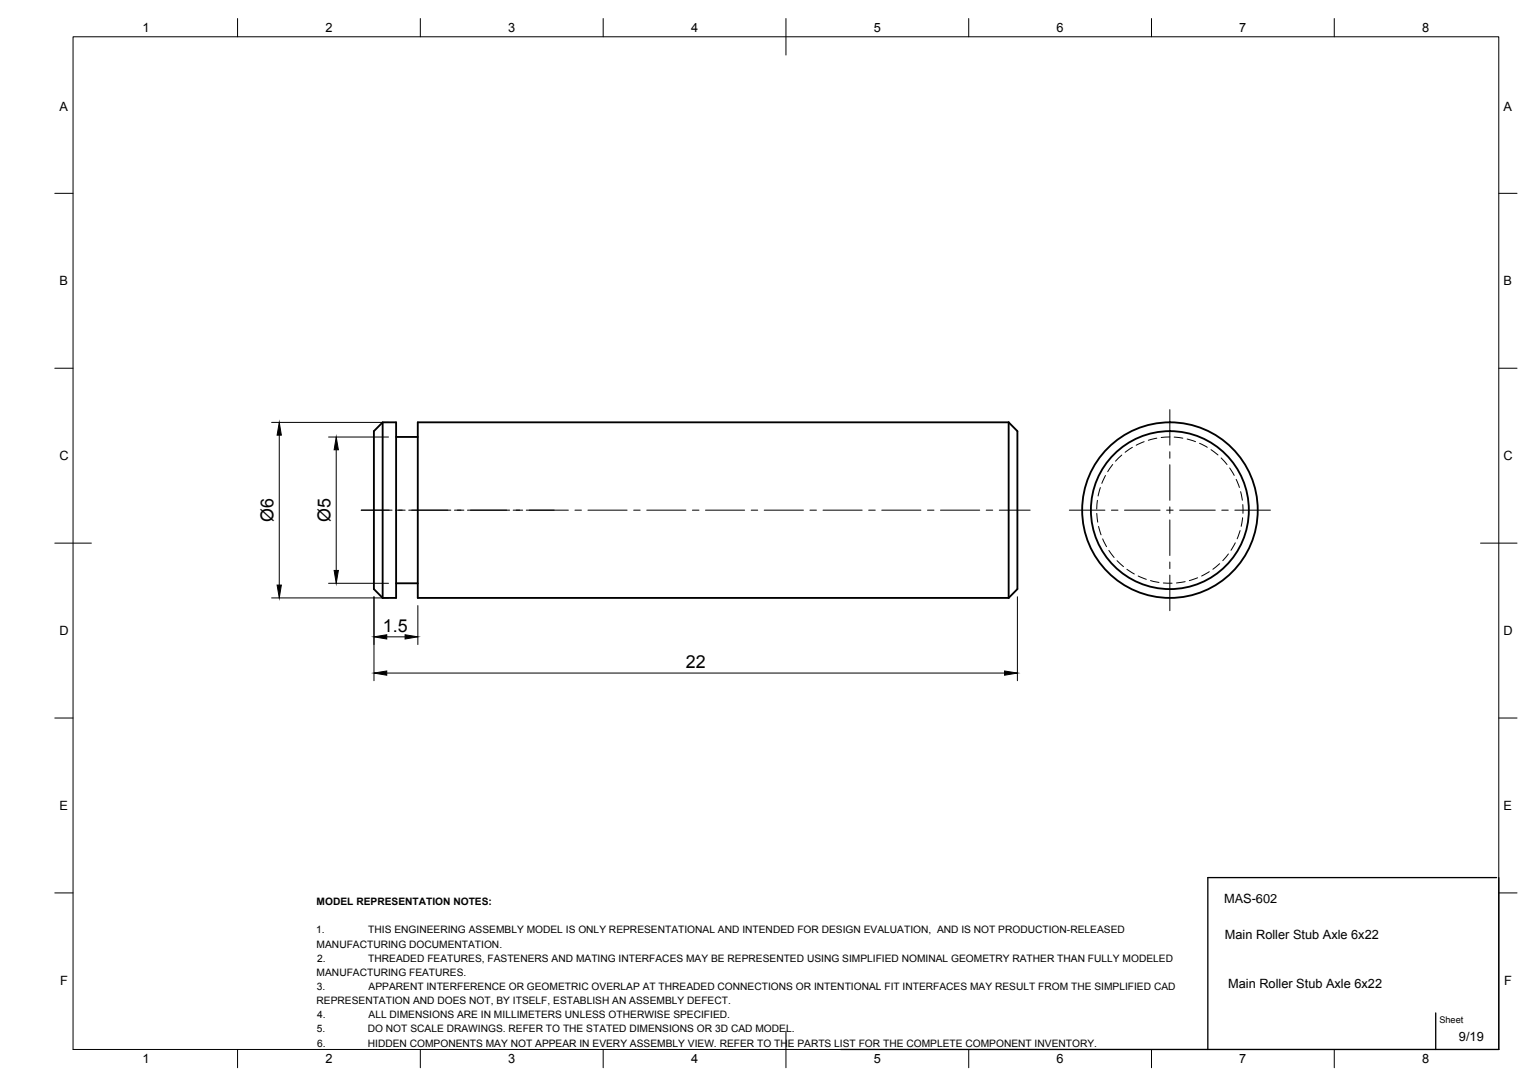
ISO-10303-21;
HEADER;
/* Generated by software containing ST-Developer
 * from STEP Tools, Inc. (www.steptools.com) 
 */

FILE_DESCRIPTION(
/* description */ (''),
/* implementation_level */ '2;1');

FILE_NAME(
/* name */ 'Main Roller Stub Axle 6x22.step',
/* time_stamp */ '2026-10-15T14:42:47-07:00',
/* author */ (''),
/* organization */ (''),
/* preprocessor_version */ 'ST-DEVELOPER v20.2',
/* originating_system */ 'Autodesk Translation Framework v15.15.0.0',
/* authorisation */ '');

FILE_SCHEMA (('AUTOMOTIVE_DESIGN { 1 0 10303 214 3 1 1 }'));
ENDSEC;

DATA;
#10=MECHANICAL_DESIGN_GEOMETRIC_PRESENTATION_REPRESENTATION('',(#246),#85789);
#185=CONICAL_SURFACE('',#10744,0.285,0.785398163397449);
#186=CONICAL_SURFACE('',#10756,0.285,0.785398163397444);
#210=SHAPE_REPRESENTATION_RELATIONSHIP('SRR','None',#85875,#228);
#228=ADVANCED_BREP_SHAPE_REPRESENTATION('',(#264),#85783);
#246=STYLED_ITEM('',(#85974),#264);
#264=MANIFOLD_SOLID_BREP('Body1',#9893);
#469=FACE_BOUND('',#3398,.T.);
#470=FACE_BOUND('',#3401,.T.);
#1167=PLANE('',#10742);
#1168=PLANE('',#10748);
#1169=PLANE('',#10752);
#1170=PLANE('',#10758);
#1650=LINE('',#77818,#2186);
#1651=LINE('',#77822,#2187);
#1652=LINE('',#77829,#2188);
#1653=LINE('',#77836,#2189);
#1654=LINE('',#77839,#2190);
#2186=VECTOR('',#12706,0.285);
#2187=VECTOR('',#12711,0.3);
#2188=VECTOR('',#12720,0.25);
#2189=VECTOR('',#12729,0.3);
#2190=VECTOR('',#12732,0.285);
#2358=CYLINDRICAL_SURFACE('',#10746,0.3);
#2359=CYLINDRICAL_SURFACE('',#10750,0.25);
#2360=CYLINDRICAL_SURFACE('',#10754,0.3);
#2810=FACE_OUTER_BOUND('',#3394,.T.);
#2811=FACE_OUTER_BOUND('',#3395,.T.);
#2812=FACE_OUTER_BOUND('',#3396,.T.);
#2813=FACE_OUTER_BOUND('',#3397,.T.);
#2814=FACE_OUTER_BOUND('',#3399,.T.);
#2815=FACE_OUTER_BOUND('',#3400,.T.);
#2816=FACE_OUTER_BOUND('',#3402,.T.);
#2817=FACE_OUTER_BOUND('',#3403,.T.);
#2818=FACE_OUTER_BOUND('',#3404,.T.);
#3394=EDGE_LOOP('',(#8837));
#3395=EDGE_LOOP('',(#8838,#8839,#8840,#8841));
#3396=EDGE_LOOP('',(#8842,#8843,#8844,#8845));
#3397=EDGE_LOOP('',(#8846));
#3398=EDGE_LOOP('',(#8847));
#3399=EDGE_LOOP('',(#8848,#8849,#8850,#8851));
#3400=EDGE_LOOP('',(#8852));
#3401=EDGE_LOOP('',(#8853));
#3402=EDGE_LOOP('',(#8854,#8855,#8856,#8857));
#3403=EDGE_LOOP('',(#8858,#8859,#8860,#8861));
#3404=EDGE_LOOP('',(#8862));
#3804=CIRCLE('',#10743,0.27);
#3805=CIRCLE('',#10745,0.3);
#3806=CIRCLE('',#10747,0.3);
#3807=CIRCLE('',#10749,0.25);
#3808=CIRCLE('',#10751,0.25);
#3809=CIRCLE('',#10753,0.3);
#3810=CIRCLE('',#10755,0.3);
#3811=CIRCLE('',#10757,0.27);
#4741=VERTEX_POINT('',#77813);
#4742=VERTEX_POINT('',#77816);
#4743=VERTEX_POINT('',#77820);
#4744=VERTEX_POINT('',#77824);
#4745=VERTEX_POINT('',#77827);
#4746=VERTEX_POINT('',#77831);
#4747=VERTEX_POINT('',#77834);
#4748=VERTEX_POINT('',#77838);
#6146=EDGE_CURVE('',#4741,#4741,#3804,.T.);
#6147=EDGE_CURVE('',#4742,#4742,#3805,.T.);
#6148=EDGE_CURVE('',#4742,#4741,#1650,.T.);
#6149=EDGE_CURVE('',#4743,#4743,#3806,.T.);
#6150=EDGE_CURVE('',#4743,#4742,#1651,.T.);
#6151=EDGE_CURVE('',#4744,#4744,#3807,.T.);
#6152=EDGE_CURVE('',#4745,#4745,#3808,.T.);
#6153=EDGE_CURVE('',#4745,#4744,#1652,.T.);
#6154=EDGE_CURVE('',#4746,#4746,#3809,.T.);
#6155=EDGE_CURVE('',#4747,#4747,#3810,.T.);
#6156=EDGE_CURVE('',#4747,#4746,#1653,.T.);
#6157=EDGE_CURVE('',#4747,#4748,#1654,.T.);
#6158=EDGE_CURVE('',#4748,#4748,#3811,.T.);
#8837=ORIENTED_EDGE('',*,*,#6146,.F.);
#8838=ORIENTED_EDGE('',*,*,#6147,.F.);
#8839=ORIENTED_EDGE('',*,*,#6148,.T.);
#8840=ORIENTED_EDGE('',*,*,#6146,.T.);
#8841=ORIENTED_EDGE('',*,*,#6148,.F.);
#8842=ORIENTED_EDGE('',*,*,#6149,.F.);
#8843=ORIENTED_EDGE('',*,*,#6150,.T.);
#8844=ORIENTED_EDGE('',*,*,#6147,.T.);
#8845=ORIENTED_EDGE('',*,*,#6150,.F.);
#8846=ORIENTED_EDGE('',*,*,#6149,.T.);
#8847=ORIENTED_EDGE('',*,*,#6151,.F.);
#8848=ORIENTED_EDGE('',*,*,#6152,.F.);
#8849=ORIENTED_EDGE('',*,*,#6153,.T.);
#8850=ORIENTED_EDGE('',*,*,#6151,.T.);
#8851=ORIENTED_EDGE('',*,*,#6153,.F.);
#8852=ORIENTED_EDGE('',*,*,#6154,.F.);
#8853=ORIENTED_EDGE('',*,*,#6152,.T.);
#8854=ORIENTED_EDGE('',*,*,#6155,.F.);
#8855=ORIENTED_EDGE('',*,*,#6156,.T.);
#8856=ORIENTED_EDGE('',*,*,#6154,.T.);
#8857=ORIENTED_EDGE('',*,*,#6156,.F.);
#8858=ORIENTED_EDGE('',*,*,#6155,.T.);
#8859=ORIENTED_EDGE('',*,*,#6157,.T.);
#8860=ORIENTED_EDGE('',*,*,#6158,.F.);
#8861=ORIENTED_EDGE('',*,*,#6157,.F.);
#8862=ORIENTED_EDGE('',*,*,#6158,.T.);
#9788=ADVANCED_FACE('',(#2810),#1167,.T.);
#9789=ADVANCED_FACE('',(#2811),#185,.T.);
#9790=ADVANCED_FACE('',(#2812),#2358,.T.);
#9791=ADVANCED_FACE('',(#2813,#469),#1168,.T.);
#9792=ADVANCED_FACE('',(#2814),#2359,.T.);
#9793=ADVANCED_FACE('',(#2815,#470),#1169,.T.);
#9794=ADVANCED_FACE('',(#2816),#2360,.T.);
#9795=ADVANCED_FACE('',(#2817),#186,.T.);
#9796=ADVANCED_FACE('',(#2818),#1170,.T.);
#9893=CLOSED_SHELL('',(#9788,#9789,#9790,#9791,#9792,#9793,#9794,#9795,
#9796));
#10741=AXIS2_PLACEMENT_3D('',#77811,#12696,#12697);
#10742=AXIS2_PLACEMENT_3D('',#77812,#12698,#12699);
#10743=AXIS2_PLACEMENT_3D('',#77814,#12700,#12701);
#10744=AXIS2_PLACEMENT_3D('',#77815,#12702,#12703);
#10745=AXIS2_PLACEMENT_3D('',#77817,#12704,#12705);
#10746=AXIS2_PLACEMENT_3D('',#77819,#12707,#12708);
#10747=AXIS2_PLACEMENT_3D('',#77821,#12709,#12710);
#10748=AXIS2_PLACEMENT_3D('',#77823,#12712,#12713);
#10749=AXIS2_PLACEMENT_3D('',#77825,#12714,#12715);
#10750=AXIS2_PLACEMENT_3D('',#77826,#12716,#12717);
#10751=AXIS2_PLACEMENT_3D('',#77828,#12718,#12719);
#10752=AXIS2_PLACEMENT_3D('',#77830,#12721,#12722);
#10753=AXIS2_PLACEMENT_3D('',#77832,#12723,#12724);
#10754=AXIS2_PLACEMENT_3D('',#77833,#12725,#12726);
#10755=AXIS2_PLACEMENT_3D('',#77835,#12727,#12728);
#10756=AXIS2_PLACEMENT_3D('',#77837,#12730,#12731);
#10757=AXIS2_PLACEMENT_3D('',#77840,#12733,#12734);
#10758=AXIS2_PLACEMENT_3D('',#77841,#12735,#12736);
#12696=DIRECTION('axis',(0.,0.,1.));
#12697=DIRECTION('refdir',(1.,0.,0.));
#12698=DIRECTION('center_axis',(-1.,0.,0.));
#12699=DIRECTION('ref_axis',(0.,0.,1.));
#12700=DIRECTION('center_axis',(1.,0.,0.));
#12701=DIRECTION('ref_axis',(0.,0.,-1.));
#12702=DIRECTION('center_axis',(1.,0.,0.));
#12703=DIRECTION('ref_axis',(0.,1.,0.));
#12704=DIRECTION('center_axis',(1.,0.,0.));
#12705=DIRECTION('ref_axis',(0.,0.,-1.));
#12706=DIRECTION('',(-0.707106781186547,0.707106781186548,8.65956056235494E-17));
#12707=DIRECTION('center_axis',(1.,0.,0.));
#12708=DIRECTION('ref_axis',(0.,1.,0.));
#12709=DIRECTION('center_axis',(1.,0.,0.));
#12710=DIRECTION('ref_axis',(0.,0.,-1.));
#12711=DIRECTION('',(-1.,0.,0.));
#12712=DIRECTION('center_axis',(1.,0.,0.));
#12713=DIRECTION('ref_axis',(0.,0.,-1.));
#12714=DIRECTION('center_axis',(1.,0.,0.));
#12715=DIRECTION('ref_axis',(0.,0.,-1.));
#12716=DIRECTION('center_axis',(1.,0.,0.));
#12717=DIRECTION('ref_axis',(0.,1.,0.));
#12718=DIRECTION('center_axis',(1.,0.,0.));
#12719=DIRECTION('ref_axis',(0.,0.,-1.));
#12720=DIRECTION('',(-1.,0.,0.));
#12721=DIRECTION('center_axis',(-1.,0.,0.));
#12722=DIRECTION('ref_axis',(0.,0.,1.));
#12723=DIRECTION('center_axis',(1.,0.,0.));
#12724=DIRECTION('ref_axis',(0.,0.,-1.));
#12725=DIRECTION('center_axis',(1.,0.,0.));
#12726=DIRECTION('ref_axis',(0.,1.,0.));
#12727=DIRECTION('center_axis',(1.,0.,0.));
#12728=DIRECTION('ref_axis',(0.,0.,-1.));
#12729=DIRECTION('',(-1.,0.,0.));
#12730=DIRECTION('center_axis',(-1.,0.,0.));
#12731=DIRECTION('ref_axis',(0.,1.,0.));
#12732=DIRECTION('',(0.707106781186551,0.707106781186544,-8.6595605623549E-17));
#12733=DIRECTION('center_axis',(1.,0.,0.));
#12734=DIRECTION('ref_axis',(0.,0.,-1.));
#12735=DIRECTION('center_axis',(1.,0.,0.));
#12736=DIRECTION('ref_axis',(0.,0.,-1.));
#77811=CARTESIAN_POINT('',(0.,0.,0.));
#77812=CARTESIAN_POINT('Origin',(0.55,0.27,0.));
#77813=CARTESIAN_POINT('',(0.55,-0.27,-3.30654635769785E-17));
#77814=CARTESIAN_POINT('Origin',(0.55,0.,0.));
#77815=CARTESIAN_POINT('Origin',(0.565,0.,0.));
#77816=CARTESIAN_POINT('',(0.58,-0.3,-3.67394039744206E-17));
#77817=CARTESIAN_POINT('Origin',(0.58,0.,0.));
#77818=CARTESIAN_POINT('',(0.565,-0.285,-3.49024337756996E-17));
#77819=CARTESIAN_POINT('Origin',(1.59,0.,0.));
#77820=CARTESIAN_POINT('',(2.6,-0.3,-3.67394039744206E-17));
#77821=CARTESIAN_POINT('Origin',(2.6,0.,0.));
#77822=CARTESIAN_POINT('',(1.59,-0.3,-3.67394039744206E-17));
#77823=CARTESIAN_POINT('Origin',(2.6,0.25,0.));
#77824=CARTESIAN_POINT('',(2.6,-0.25,-3.06161699786838E-17));
#77825=CARTESIAN_POINT('Origin',(2.6,0.,0.));
#77826=CARTESIAN_POINT('Origin',(2.637,0.,0.));
#77827=CARTESIAN_POINT('',(2.674,-0.25,-3.06161699786838E-17));
#77828=CARTESIAN_POINT('Origin',(2.674,0.,0.));
#77829=CARTESIAN_POINT('',(2.637,-0.25,-3.06161699786838E-17));
#77830=CARTESIAN_POINT('Origin',(2.674,0.3,0.));
#77831=CARTESIAN_POINT('',(2.674,-0.3,-3.67394039744206E-17));
#77832=CARTESIAN_POINT('Origin',(2.674,0.,0.));
#77833=CARTESIAN_POINT('Origin',(2.697,0.,0.));
#77834=CARTESIAN_POINT('',(2.72,-0.3,-3.67394039744206E-17));
#77835=CARTESIAN_POINT('Origin',(2.72,0.,0.));
#77836=CARTESIAN_POINT('',(2.697,-0.3,-3.67394039744206E-17));
#77837=CARTESIAN_POINT('Origin',(2.735,0.,0.));
#77838=CARTESIAN_POINT('',(2.75,-0.27,-3.30654635769785E-17));
#77839=CARTESIAN_POINT('',(2.735,-0.285,3.49024337756996E-17));
#77840=CARTESIAN_POINT('Origin',(2.75,0.,0.));
#77841=CARTESIAN_POINT('Origin',(2.75,0.,0.));
#85763=UNCERTAINTY_MEASURE_WITH_UNIT(LENGTH_MEASURE(0.001),#85790,
'DISTANCE_ACCURACY_VALUE',
'Maximum model space distance between geometric entities at asserted c
onnectivities');
#85769=UNCERTAINTY_MEASURE_WITH_UNIT(LENGTH_MEASURE(0.001),#85790,
'DISTANCE_ACCURACY_VALUE',
'Maximum model space distance between geometric entities at asserted c
onnectivities');
#85783=(
GEOMETRIC_REPRESENTATION_CONTEXT(3)
GLOBAL_UNCERTAINTY_ASSIGNED_CONTEXT((#85763))
GLOBAL_UNIT_ASSIGNED_CONTEXT((#85790,#85792,#85793))
REPRESENTATION_CONTEXT('','3D')
);
#85789=(
GEOMETRIC_REPRESENTATION_CONTEXT(3)
GLOBAL_UNCERTAINTY_ASSIGNED_CONTEXT((#85769))
GLOBAL_UNIT_ASSIGNED_CONTEXT((#85790,#85792,#85793))
REPRESENTATION_CONTEXT('','3D')
);
#85790=(
LENGTH_UNIT()
NAMED_UNIT(*)
SI_UNIT(.CENTI.,.METRE.)
);
#85792=(
NAMED_UNIT(*)
PLANE_ANGLE_UNIT()
SI_UNIT($,.RADIAN.)
);
#85793=(
NAMED_UNIT(*)
SI_UNIT($,.STERADIAN.)
SOLID_ANGLE_UNIT()
);
#85807=SHAPE_DEFINITION_REPRESENTATION(#85826,#85875);
#85826=PRODUCT_DEFINITION_SHAPE('',$,#85895);
#85875=SHAPE_REPRESENTATION('',(#10741),#85783);
#85881=PRODUCT_DEFINITION_CONTEXT('part definition',#85940,'design');
#85895=PRODUCT_DEFINITION('Main Roller Stub Axle 6x22',
'Main Roller Stub Axle 6x22',#85914,#85881);
#85914=PRODUCT_DEFINITION_FORMATION('',$,#85955);
#85940=APPLICATION_CONTEXT(
'Core Data for Automotive Mechanical Design Process');
#85941=PRODUCT_CONTEXT('part definition',#85940,'mechanical');
#85955=PRODUCT('Main Roller Stub Axle 6x22',
'Main Roller Stub Axle 6x22',$,(#85941));
#85974=PRESENTATION_STYLE_ASSIGNMENT((#85992));
#85992=SURFACE_STYLE_USAGE(.BOTH.,#86010);
#86010=SURFACE_SIDE_STYLE('',(#86028));
#86028=SURFACE_STYLE_FILL_AREA(#86046);
#86046=FILL_AREA_STYLE('Opaque(216,219,224)',(#86064));
#86064=FILL_AREA_STYLE_COLOUR('Opaque(216,219,224)',#86082);
#86082=COLOUR_RGB('Opaque(216,219,224)', 0.66274510, 0.83137255, 0.94901961);
ENDSEC;
END-ISO-10303-21;
